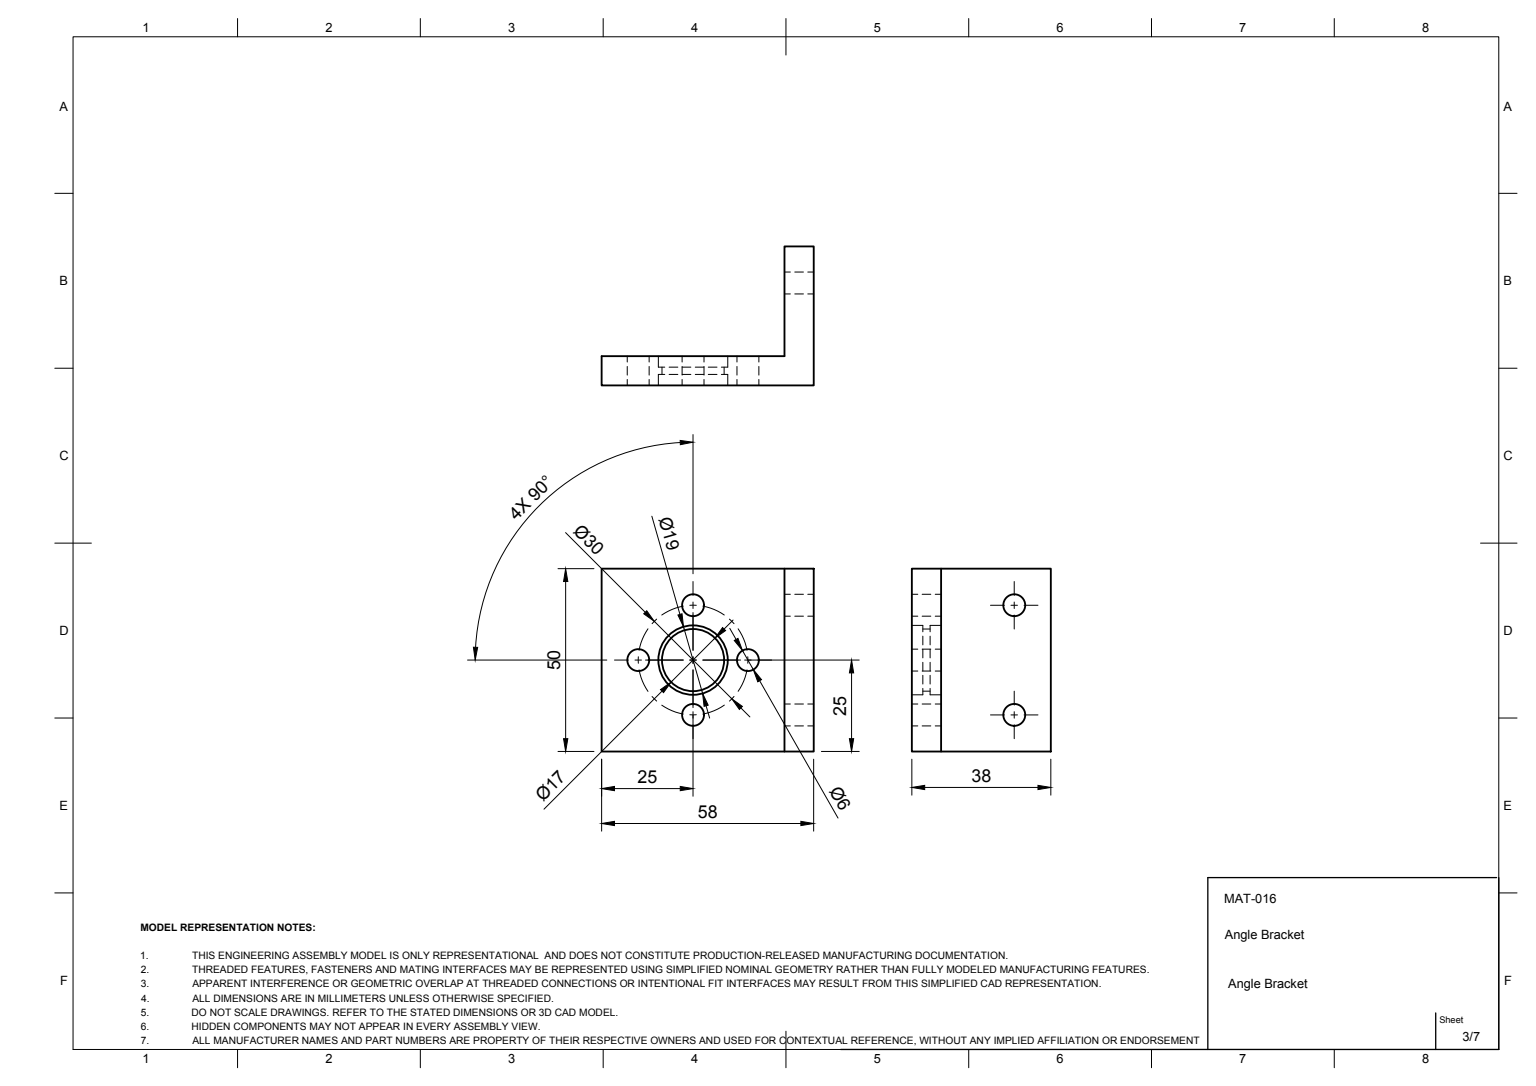
ISO-10303-21;
HEADER;
/* Generated by software containing ST-Developer
 * from STEP Tools, Inc. (www.steptools.com) 
 */

FILE_DESCRIPTION(
/* description */ ('STEP AP214'),
/* implementation_level */ '2;1');

FILE_NAME(
/* name */ 'Angle Bracket.step',
/* time_stamp */ '2026-11-14T06:10:26-08:00',
/* author */ (''),
/* organization */ (''),
/* preprocessor_version */ 'ST-DEVELOPER v20.2',
/* originating_system */ 'Autodesk Translation Framework v15.17.0.0',
/* authorisation */ '');

FILE_SCHEMA (('AUTOMOTIVE_DESIGN { 1 0 10303 214 3 1 1 }'));
ENDSEC;

DATA;
#10=MECHANICAL_DESIGN_GEOMETRIC_PRESENTATION_REPRESENTATION('',(#164),#10413);
#148=SHAPE_REPRESENTATION_RELATIONSHIP('SRR','None',#10453,#156);
#156=ADVANCED_BREP_SHAPE_REPRESENTATION('',(#172),#10405);
#164=STYLED_ITEM('',(#10502),#172);
#172=MANIFOLD_SOLID_BREP('Body1',#5299);
#180=FACE_BOUND('',#575,.T.);
#181=FACE_BOUND('',#576,.T.);
#182=FACE_BOUND('',#577,.T.);
#183=FACE_BOUND('',#578,.T.);
#184=FACE_BOUND('',#579,.T.);
#185=FACE_BOUND('',#581,.T.);
#186=FACE_BOUND('',#582,.T.);
#187=FACE_BOUND('',#583,.T.);
#188=FACE_BOUND('',#584,.T.);
#189=FACE_BOUND('',#585,.T.);
#190=FACE_BOUND('',#589,.T.);
#191=FACE_BOUND('',#591,.T.);
#192=FACE_BOUND('',#594,.T.);
#193=FACE_BOUND('',#595,.T.);
#194=FACE_BOUND('',#597,.T.);
#195=FACE_BOUND('',#598,.T.);
#219=PLANE('',#5425);
#220=PLANE('',#5426);
#221=PLANE('',#5427);
#222=PLANE('',#5428);
#223=PLANE('',#5429);
#224=PLANE('',#5430);
#225=PLANE('',#5431);
#226=PLANE('',#5432);
#227=PLANE('',#5433);
#228=PLANE('',#5434);
#275=FACE_OUTER_BOUND('',#565,.T.);
#276=FACE_OUTER_BOUND('',#566,.T.);
#277=FACE_OUTER_BOUND('',#567,.T.);
#278=FACE_OUTER_BOUND('',#568,.T.);
#279=FACE_OUTER_BOUND('',#569,.T.);
#280=FACE_OUTER_BOUND('',#570,.T.);
#281=FACE_OUTER_BOUND('',#571,.T.);
#282=FACE_OUTER_BOUND('',#572,.T.);
#283=FACE_OUTER_BOUND('',#573,.T.);
#284=FACE_OUTER_BOUND('',#574,.T.);
#285=FACE_OUTER_BOUND('',#580,.T.);
#286=FACE_OUTER_BOUND('',#586,.T.);
#287=FACE_OUTER_BOUND('',#587,.T.);
#288=FACE_OUTER_BOUND('',#588,.T.);
#289=FACE_OUTER_BOUND('',#590,.T.);
#290=FACE_OUTER_BOUND('',#592,.T.);
#291=FACE_OUTER_BOUND('',#593,.T.);
#292=FACE_OUTER_BOUND('',#596,.T.);
#293=FACE_OUTER_BOUND('',#599,.T.);
#565=EDGE_LOOP('',(#3222,#3223,#3224,#3225));
#566=EDGE_LOOP('',(#3226,#3227,#3228,#3229));
#567=EDGE_LOOP('',(#3230,#3231,#3232,#3233));
#568=EDGE_LOOP('',(#3234,#3235,#3236,#3237));
#569=EDGE_LOOP('',(#3238,#3239,#3240,#3241));
#570=EDGE_LOOP('',(#3242,#3243,#3244,#3245));
#571=EDGE_LOOP('',(#3246,#3247,#3248,#3249));
#572=EDGE_LOOP('',(#3250,#3251,#3252,#3253));
#573=EDGE_LOOP('',(#3254,#3255,#3256,#3257));
#574=EDGE_LOOP('',(#3258,#3259,#3260,#3261));
#575=EDGE_LOOP('',(#3262));
#576=EDGE_LOOP('',(#3263));
#577=EDGE_LOOP('',(#3264));
#578=EDGE_LOOP('',(#3265));
#579=EDGE_LOOP('',(#3266));
#580=EDGE_LOOP('',(#3267,#3268,#3269,#3270));
#581=EDGE_LOOP('',(#3271));
#582=EDGE_LOOP('',(#3272));
#583=EDGE_LOOP('',(#3273));
#584=EDGE_LOOP('',(#3274));
#585=EDGE_LOOP('',(#3275));
#586=EDGE_LOOP('',(#3276,#3277,#3278,#3279,#3280,#3281));
#587=EDGE_LOOP('',(#3282,#3283,#3284,#3285,#3286,#3287));
#588=EDGE_LOOP('',(#3288));
#589=EDGE_LOOP('',(#3289));
#590=EDGE_LOOP('',(#3290));
#591=EDGE_LOOP('',(#3291));
#592=EDGE_LOOP('',(#3292,#3293,#3294,#3295));
#593=EDGE_LOOP('',(#3296,#3297,#3298,#3299));
#594=EDGE_LOOP('',(#3300));
#595=EDGE_LOOP('',(#3301));
#596=EDGE_LOOP('',(#3302,#3303,#3304,#3305));
#597=EDGE_LOOP('',(#3306));
#598=EDGE_LOOP('',(#3307));
#599=EDGE_LOOP('',(#3308,#3309,#3310,#3311));
#894=LINE('',#7955,#1185);
#895=LINE('',#7961,#1186);
#896=LINE('',#7967,#1187);
#897=LINE('',#7973,#1188);
#898=LINE('',#7979,#1189);
#899=LINE('',#7985,#1190);
#900=LINE('',#7991,#1191);
#901=LINE('',#7997,#1192);
#902=LINE('',#8003,#1193);
#903=LINE('',#8008,#1194);
#904=LINE('',#8010,#1195);
#905=LINE('',#8012,#1196);
#906=LINE('',#8013,#1197);
#907=LINE('',#8017,#1198);
#908=LINE('',#8019,#1199);
#909=LINE('',#8021,#1200);
#910=LINE('',#8022,#1201);
#911=LINE('',#8024,#1202);
#912=LINE('',#8026,#1203);
#913=LINE('',#8028,#1204);
#914=LINE('',#8029,#1205);
#915=LINE('',#8031,#1206);
#916=LINE('',#8033,#1207);
#917=LINE('',#8035,#1208);
#918=LINE('',#8036,#1209);
#919=LINE('',#8041,#1210);
#920=LINE('',#8043,#1211);
#1185=VECTOR('',#6158,3.);
#1186=VECTOR('',#6165,3.);
#1187=VECTOR('',#6172,8.5);
#1188=VECTOR('',#6179,9.5);
#1189=VECTOR('',#6186,9.5);
#1190=VECTOR('',#6193,2.99999999999929);
#1191=VECTOR('',#6200,3.);
#1192=VECTOR('',#6207,2.99999999999976);
#1193=VECTOR('',#6214,3.);
#1194=VECTOR('',#6219,1000.);
#1195=VECTOR('',#6220,1000.);
#1196=VECTOR('',#6221,1000.);
#1197=VECTOR('',#6222,1000.);
#1198=VECTOR('',#6225,1000.);
#1199=VECTOR('',#6226,1000.);
#1200=VECTOR('',#6227,1000.);
#1201=VECTOR('',#6228,1000.);
#1202=VECTOR('',#6231,1000.);
#1203=VECTOR('',#6232,1000.);
#1204=VECTOR('',#6233,1000.);
#1205=VECTOR('',#6234,1000.);
#1206=VECTOR('',#6237,1000.);
#1207=VECTOR('',#6238,1000.);
#1208=VECTOR('',#6239,1000.);
#1209=VECTOR('',#6240,1000.);
#1210=VECTOR('',#6249,1000.);
#1211=VECTOR('',#6252,1000.);
#1476=CIRCLE('',#5399,3.);
#1477=CIRCLE('',#5400,3.);
#1478=CIRCLE('',#5402,3.);
#1479=CIRCLE('',#5403,3.);
#1480=CIRCLE('',#5405,8.5);
#1481=CIRCLE('',#5406,8.5);
#1482=CIRCLE('',#5408,9.5);
#1483=CIRCLE('',#5409,9.5);
#1484=CIRCLE('',#5411,9.5);
#1485=CIRCLE('',#5412,9.5);
#1486=CIRCLE('',#5414,2.99999999999929);
#1487=CIRCLE('',#5415,2.99999999999929);
#1488=CIRCLE('',#5417,3.);
#1489=CIRCLE('',#5418,3.);
#1490=CIRCLE('',#5420,2.99999999999976);
#1491=CIRCLE('',#5421,2.99999999999976);
#1492=CIRCLE('',#5423,3.);
#1493=CIRCLE('',#5424,3.);
#1917=VERTEX_POINT('',#7952);
#1918=VERTEX_POINT('',#7954);
#1919=VERTEX_POINT('',#7958);
#1920=VERTEX_POINT('',#7960);
#1921=VERTEX_POINT('',#7964);
#1922=VERTEX_POINT('',#7966);
#1923=VERTEX_POINT('',#7970);
#1924=VERTEX_POINT('',#7972);
#1925=VERTEX_POINT('',#7976);
#1926=VERTEX_POINT('',#7978);
#1927=VERTEX_POINT('',#7982);
#1928=VERTEX_POINT('',#7984);
#1929=VERTEX_POINT('',#7988);
#1930=VERTEX_POINT('',#7990);
#1931=VERTEX_POINT('',#7994);
#1932=VERTEX_POINT('',#7996);
#1933=VERTEX_POINT('',#8000);
#1934=VERTEX_POINT('',#8002);
#1935=VERTEX_POINT('',#8006);
#1936=VERTEX_POINT('',#8007);
#1937=VERTEX_POINT('',#8009);
#1938=VERTEX_POINT('',#8011);
#1939=VERTEX_POINT('',#8015);
#1940=VERTEX_POINT('',#8016);
#1941=VERTEX_POINT('',#8018);
#1942=VERTEX_POINT('',#8020);
#1943=VERTEX_POINT('',#8025);
#1944=VERTEX_POINT('',#8027);
#1945=VERTEX_POINT('',#8032);
#1946=VERTEX_POINT('',#8034);
#2436=EDGE_CURVE('',#1917,#1917,#1476,.T.);
#2437=EDGE_CURVE('',#1917,#1918,#894,.T.);
#2438=EDGE_CURVE('',#1918,#1918,#1477,.T.);
#2439=EDGE_CURVE('',#1919,#1919,#1478,.T.);
#2440=EDGE_CURVE('',#1919,#1920,#895,.T.);
#2441=EDGE_CURVE('',#1920,#1920,#1479,.T.);
#2442=EDGE_CURVE('',#1921,#1921,#1480,.T.);
#2443=EDGE_CURVE('',#1921,#1922,#896,.T.);
#2444=EDGE_CURVE('',#1922,#1922,#1481,.T.);
#2445=EDGE_CURVE('',#1923,#1923,#1482,.T.);
#2446=EDGE_CURVE('',#1923,#1924,#897,.T.);
#2447=EDGE_CURVE('',#1924,#1924,#1483,.T.);
#2448=EDGE_CURVE('',#1925,#1925,#1484,.T.);
#2449=EDGE_CURVE('',#1925,#1926,#898,.T.);
#2450=EDGE_CURVE('',#1926,#1926,#1485,.T.);
#2451=EDGE_CURVE('',#1927,#1927,#1486,.T.);
#2452=EDGE_CURVE('',#1927,#1928,#899,.T.);
#2453=EDGE_CURVE('',#1928,#1928,#1487,.T.);
#2454=EDGE_CURVE('',#1929,#1929,#1488,.T.);
#2455=EDGE_CURVE('',#1929,#1930,#900,.T.);
#2456=EDGE_CURVE('',#1930,#1930,#1489,.T.);
#2457=EDGE_CURVE('',#1931,#1931,#1490,.T.);
#2458=EDGE_CURVE('',#1931,#1932,#901,.T.);
#2459=EDGE_CURVE('',#1932,#1932,#1491,.T.);
#2460=EDGE_CURVE('',#1933,#1933,#1492,.T.);
#2461=EDGE_CURVE('',#1933,#1934,#902,.T.);
#2462=EDGE_CURVE('',#1934,#1934,#1493,.T.);
#2463=EDGE_CURVE('',#1935,#1936,#903,.T.);
#2464=EDGE_CURVE('',#1935,#1937,#904,.T.);
#2465=EDGE_CURVE('',#1938,#1937,#905,.T.);
#2466=EDGE_CURVE('',#1938,#1936,#906,.T.);
#2467=EDGE_CURVE('',#1939,#1940,#907,.T.);
#2468=EDGE_CURVE('',#1941,#1939,#908,.T.);
#2469=EDGE_CURVE('',#1942,#1941,#909,.T.);
#2470=EDGE_CURVE('',#1940,#1942,#910,.T.);
#2471=EDGE_CURVE('',#1940,#1938,#911,.T.);
#2472=EDGE_CURVE('',#1942,#1943,#912,.T.);
#2473=EDGE_CURVE('',#1944,#1943,#913,.T.);
#2474=EDGE_CURVE('',#1944,#1936,#914,.T.);
#2475=EDGE_CURVE('',#1939,#1937,#915,.T.);
#2476=EDGE_CURVE('',#1945,#1935,#916,.T.);
#2477=EDGE_CURVE('',#1946,#1945,#917,.T.);
#2478=EDGE_CURVE('',#1941,#1946,#918,.T.);
#2479=EDGE_CURVE('',#1943,#1946,#919,.T.);
#2480=EDGE_CURVE('',#1945,#1944,#920,.T.);
#3222=ORIENTED_EDGE('',*,*,#2436,.F.);
#3223=ORIENTED_EDGE('',*,*,#2437,.T.);
#3224=ORIENTED_EDGE('',*,*,#2438,.T.);
#3225=ORIENTED_EDGE('',*,*,#2437,.F.);
#3226=ORIENTED_EDGE('',*,*,#2439,.F.);
#3227=ORIENTED_EDGE('',*,*,#2440,.T.);
#3228=ORIENTED_EDGE('',*,*,#2441,.T.);
#3229=ORIENTED_EDGE('',*,*,#2440,.F.);
#3230=ORIENTED_EDGE('',*,*,#2442,.T.);
#3231=ORIENTED_EDGE('',*,*,#2443,.T.);
#3232=ORIENTED_EDGE('',*,*,#2444,.T.);
#3233=ORIENTED_EDGE('',*,*,#2443,.F.);
#3234=ORIENTED_EDGE('',*,*,#2445,.T.);
#3235=ORIENTED_EDGE('',*,*,#2446,.T.);
#3236=ORIENTED_EDGE('',*,*,#2447,.F.);
#3237=ORIENTED_EDGE('',*,*,#2446,.F.);
#3238=ORIENTED_EDGE('',*,*,#2448,.F.);
#3239=ORIENTED_EDGE('',*,*,#2449,.T.);
#3240=ORIENTED_EDGE('',*,*,#2450,.T.);
#3241=ORIENTED_EDGE('',*,*,#2449,.F.);
#3242=ORIENTED_EDGE('',*,*,#2451,.F.);
#3243=ORIENTED_EDGE('',*,*,#2452,.T.);
#3244=ORIENTED_EDGE('',*,*,#2453,.T.);
#3245=ORIENTED_EDGE('',*,*,#2452,.F.);
#3246=ORIENTED_EDGE('',*,*,#2454,.F.);
#3247=ORIENTED_EDGE('',*,*,#2455,.T.);
#3248=ORIENTED_EDGE('',*,*,#2456,.T.);
#3249=ORIENTED_EDGE('',*,*,#2455,.F.);
#3250=ORIENTED_EDGE('',*,*,#2457,.F.);
#3251=ORIENTED_EDGE('',*,*,#2458,.T.);
#3252=ORIENTED_EDGE('',*,*,#2459,.T.);
#3253=ORIENTED_EDGE('',*,*,#2458,.F.);
#3254=ORIENTED_EDGE('',*,*,#2460,.F.);
#3255=ORIENTED_EDGE('',*,*,#2461,.T.);
#3256=ORIENTED_EDGE('',*,*,#2462,.T.);
#3257=ORIENTED_EDGE('',*,*,#2461,.F.);
#3258=ORIENTED_EDGE('',*,*,#2463,.F.);
#3259=ORIENTED_EDGE('',*,*,#2464,.T.);
#3260=ORIENTED_EDGE('',*,*,#2465,.F.);
#3261=ORIENTED_EDGE('',*,*,#2466,.T.);
#3262=ORIENTED_EDGE('',*,*,#2462,.F.);
#3263=ORIENTED_EDGE('',*,*,#2459,.F.);
#3264=ORIENTED_EDGE('',*,*,#2456,.F.);
#3265=ORIENTED_EDGE('',*,*,#2453,.F.);
#3266=ORIENTED_EDGE('',*,*,#2450,.F.);
#3267=ORIENTED_EDGE('',*,*,#2467,.F.);
#3268=ORIENTED_EDGE('',*,*,#2468,.F.);
#3269=ORIENTED_EDGE('',*,*,#2469,.F.);
#3270=ORIENTED_EDGE('',*,*,#2470,.F.);
#3271=ORIENTED_EDGE('',*,*,#2460,.T.);
#3272=ORIENTED_EDGE('',*,*,#2457,.T.);
#3273=ORIENTED_EDGE('',*,*,#2454,.T.);
#3274=ORIENTED_EDGE('',*,*,#2451,.T.);
#3275=ORIENTED_EDGE('',*,*,#2447,.T.);
#3276=ORIENTED_EDGE('',*,*,#2466,.F.);
#3277=ORIENTED_EDGE('',*,*,#2471,.F.);
#3278=ORIENTED_EDGE('',*,*,#2470,.T.);
#3279=ORIENTED_EDGE('',*,*,#2472,.T.);
#3280=ORIENTED_EDGE('',*,*,#2473,.F.);
#3281=ORIENTED_EDGE('',*,*,#2474,.T.);
#3282=ORIENTED_EDGE('',*,*,#2468,.T.);
#3283=ORIENTED_EDGE('',*,*,#2475,.T.);
#3284=ORIENTED_EDGE('',*,*,#2464,.F.);
#3285=ORIENTED_EDGE('',*,*,#2476,.F.);
#3286=ORIENTED_EDGE('',*,*,#2477,.F.);
#3287=ORIENTED_EDGE('',*,*,#2478,.F.);
#3288=ORIENTED_EDGE('',*,*,#2448,.T.);
#3289=ORIENTED_EDGE('',*,*,#2444,.F.);
#3290=ORIENTED_EDGE('',*,*,#2445,.F.);
#3291=ORIENTED_EDGE('',*,*,#2442,.F.);
#3292=ORIENTED_EDGE('',*,*,#2467,.T.);
#3293=ORIENTED_EDGE('',*,*,#2471,.T.);
#3294=ORIENTED_EDGE('',*,*,#2465,.T.);
#3295=ORIENTED_EDGE('',*,*,#2475,.F.);
#3296=ORIENTED_EDGE('',*,*,#2478,.T.);
#3297=ORIENTED_EDGE('',*,*,#2479,.F.);
#3298=ORIENTED_EDGE('',*,*,#2472,.F.);
#3299=ORIENTED_EDGE('',*,*,#2469,.T.);
#3300=ORIENTED_EDGE('',*,*,#2436,.T.);
#3301=ORIENTED_EDGE('',*,*,#2439,.T.);
#3302=ORIENTED_EDGE('',*,*,#2463,.T.);
#3303=ORIENTED_EDGE('',*,*,#2474,.F.);
#3304=ORIENTED_EDGE('',*,*,#2480,.F.);
#3305=ORIENTED_EDGE('',*,*,#2476,.T.);
#3306=ORIENTED_EDGE('',*,*,#2438,.F.);
#3307=ORIENTED_EDGE('',*,*,#2441,.F.);
#3308=ORIENTED_EDGE('',*,*,#2479,.T.);
#3309=ORIENTED_EDGE('',*,*,#2477,.T.);
#3310=ORIENTED_EDGE('',*,*,#2480,.T.);
#3311=ORIENTED_EDGE('',*,*,#2473,.T.);
#4794=CYLINDRICAL_SURFACE('',#5398,3.);
#4795=CYLINDRICAL_SURFACE('',#5401,3.);
#4796=CYLINDRICAL_SURFACE('',#5404,8.5);
#4797=CYLINDRICAL_SURFACE('',#5407,9.5);
#4798=CYLINDRICAL_SURFACE('',#5410,9.5);
#4799=CYLINDRICAL_SURFACE('',#5413,2.99999999999929);
#4800=CYLINDRICAL_SURFACE('',#5416,3.);
#4801=CYLINDRICAL_SURFACE('',#5419,2.99999999999976);
#4802=CYLINDRICAL_SURFACE('',#5422,3.);
#5009=ADVANCED_FACE('',(#275),#4794,.F.);
#5010=ADVANCED_FACE('',(#276),#4795,.F.);
#5011=ADVANCED_FACE('',(#277),#4796,.F.);
#5012=ADVANCED_FACE('',(#278),#4797,.F.);
#5013=ADVANCED_FACE('',(#279),#4798,.F.);
#5014=ADVANCED_FACE('',(#280),#4799,.F.);
#5015=ADVANCED_FACE('',(#281),#4800,.F.);
#5016=ADVANCED_FACE('',(#282),#4801,.F.);
#5017=ADVANCED_FACE('',(#283),#4802,.F.);
#5018=ADVANCED_FACE('',(#284,#180,#181,#182,#183,#184),#219,.F.);
#5019=ADVANCED_FACE('',(#285,#185,#186,#187,#188,#189),#220,.T.);
#5020=ADVANCED_FACE('',(#286),#221,.F.);
#5021=ADVANCED_FACE('',(#287),#222,.F.);
#5022=ADVANCED_FACE('',(#288,#190),#223,.T.);
#5023=ADVANCED_FACE('',(#289,#191),#224,.T.);
#5024=ADVANCED_FACE('',(#290),#225,.F.);
#5025=ADVANCED_FACE('',(#291,#192,#193),#226,.T.);
#5026=ADVANCED_FACE('',(#292,#194,#195),#227,.F.);
#5027=ADVANCED_FACE('',(#293),#228,.F.);
#5299=CLOSED_SHELL('',(#5009,#5010,#5011,#5012,#5013,#5014,#5015,#5016,
#5017,#5018,#5019,#5020,#5021,#5022,#5023,#5024,#5025,#5026,#5027));
#5397=AXIS2_PLACEMENT_3D('',#7950,#6152,#6153);
#5398=AXIS2_PLACEMENT_3D('',#7951,#6154,#6155);
#5399=AXIS2_PLACEMENT_3D('',#7953,#6156,#6157);
#5400=AXIS2_PLACEMENT_3D('',#7956,#6159,#6160);
#5401=AXIS2_PLACEMENT_3D('',#7957,#6161,#6162);
#5402=AXIS2_PLACEMENT_3D('',#7959,#6163,#6164);
#5403=AXIS2_PLACEMENT_3D('',#7962,#6166,#6167);
#5404=AXIS2_PLACEMENT_3D('',#7963,#6168,#6169);
#5405=AXIS2_PLACEMENT_3D('',#7965,#6170,#6171);
#5406=AXIS2_PLACEMENT_3D('',#7968,#6173,#6174);
#5407=AXIS2_PLACEMENT_3D('',#7969,#6175,#6176);
#5408=AXIS2_PLACEMENT_3D('',#7971,#6177,#6178);
#5409=AXIS2_PLACEMENT_3D('',#7974,#6180,#6181);
#5410=AXIS2_PLACEMENT_3D('',#7975,#6182,#6183);
#5411=AXIS2_PLACEMENT_3D('',#7977,#6184,#6185);
#5412=AXIS2_PLACEMENT_3D('',#7980,#6187,#6188);
#5413=AXIS2_PLACEMENT_3D('',#7981,#6189,#6190);
#5414=AXIS2_PLACEMENT_3D('',#7983,#6191,#6192);
#5415=AXIS2_PLACEMENT_3D('',#7986,#6194,#6195);
#5416=AXIS2_PLACEMENT_3D('',#7987,#6196,#6197);
#5417=AXIS2_PLACEMENT_3D('',#7989,#6198,#6199);
#5418=AXIS2_PLACEMENT_3D('',#7992,#6201,#6202);
#5419=AXIS2_PLACEMENT_3D('',#7993,#6203,#6204);
#5420=AXIS2_PLACEMENT_3D('',#7995,#6205,#6206);
#5421=AXIS2_PLACEMENT_3D('',#7998,#6208,#6209);
#5422=AXIS2_PLACEMENT_3D('',#7999,#6210,#6211);
#5423=AXIS2_PLACEMENT_3D('',#8001,#6212,#6213);
#5424=AXIS2_PLACEMENT_3D('',#8004,#6215,#6216);
#5425=AXIS2_PLACEMENT_3D('',#8005,#6217,#6218);
#5426=AXIS2_PLACEMENT_3D('',#8014,#6223,#6224);
#5427=AXIS2_PLACEMENT_3D('',#8023,#6229,#6230);
#5428=AXIS2_PLACEMENT_3D('',#8030,#6235,#6236);
#5429=AXIS2_PLACEMENT_3D('',#8037,#6241,#6242);
#5430=AXIS2_PLACEMENT_3D('',#8038,#6243,#6244);
#5431=AXIS2_PLACEMENT_3D('',#8039,#6245,#6246);
#5432=AXIS2_PLACEMENT_3D('',#8040,#6247,#6248);
#5433=AXIS2_PLACEMENT_3D('',#8042,#6250,#6251);
#5434=AXIS2_PLACEMENT_3D('',#8044,#6253,#6254);
#6152=DIRECTION('axis',(0.,0.,1.));
#6153=DIRECTION('refdir',(1.,0.,0.));
#6154=DIRECTION('center_axis',(-1.,0.,0.));
#6155=DIRECTION('ref_axis',(0.,0.,1.));
#6156=DIRECTION('center_axis',(-1.,0.,0.));
#6157=DIRECTION('ref_axis',(0.,0.,1.));
#6158=DIRECTION('',(-1.,0.,0.));
#6159=DIRECTION('center_axis',(-1.,0.,0.));
#6160=DIRECTION('ref_axis',(0.,0.,1.));
#6161=DIRECTION('center_axis',(-1.,0.,0.));
#6162=DIRECTION('ref_axis',(0.,0.,1.));
#6163=DIRECTION('center_axis',(-1.,0.,0.));
#6164=DIRECTION('ref_axis',(0.,0.,1.));
#6165=DIRECTION('',(-1.,0.,0.));
#6166=DIRECTION('center_axis',(-1.,0.,0.));
#6167=DIRECTION('ref_axis',(0.,0.,1.));
#6168=DIRECTION('center_axis',(0.,0.,1.));
#6169=DIRECTION('ref_axis',(1.,0.,0.));
#6170=DIRECTION('center_axis',(0.,0.,-1.));
#6171=DIRECTION('ref_axis',(-1.,0.,0.));
#6172=DIRECTION('',(0.,0.,1.));
#6173=DIRECTION('center_axis',(0.,0.,1.));
#6174=DIRECTION('ref_axis',(1.,0.,0.));
#6175=DIRECTION('center_axis',(0.,0.,-1.));
#6176=DIRECTION('ref_axis',(-1.,0.,0.));
#6177=DIRECTION('center_axis',(0.,0.,1.));
#6178=DIRECTION('ref_axis',(1.,0.,0.));
#6179=DIRECTION('',(0.,0.,-1.));
#6180=DIRECTION('center_axis',(0.,0.,1.));
#6181=DIRECTION('ref_axis',(1.,0.,0.));
#6182=DIRECTION('center_axis',(0.,0.,1.));
#6183=DIRECTION('ref_axis',(1.,0.,0.));
#6184=DIRECTION('center_axis',(0.,0.,1.));
#6185=DIRECTION('ref_axis',(1.,0.,0.));
#6186=DIRECTION('',(0.,0.,1.));
#6187=DIRECTION('center_axis',(0.,0.,1.));
#6188=DIRECTION('ref_axis',(1.,0.,0.));
#6189=DIRECTION('center_axis',(0.,0.,1.));
#6190=DIRECTION('ref_axis',(1.,0.,0.));
#6191=DIRECTION('center_axis',(0.,0.,1.));
#6192=DIRECTION('ref_axis',(1.,0.,0.));
#6193=DIRECTION('',(0.,0.,1.));
#6194=DIRECTION('center_axis',(0.,0.,1.));
#6195=DIRECTION('ref_axis',(1.,0.,0.));
#6196=DIRECTION('center_axis',(0.,0.,1.));
#6197=DIRECTION('ref_axis',(1.,0.,0.));
#6198=DIRECTION('center_axis',(0.,0.,1.));
#6199=DIRECTION('ref_axis',(1.,0.,0.));
#6200=DIRECTION('',(0.,0.,1.));
#6201=DIRECTION('center_axis',(0.,0.,1.));
#6202=DIRECTION('ref_axis',(1.,0.,0.));
#6203=DIRECTION('center_axis',(0.,0.,1.));
#6204=DIRECTION('ref_axis',(1.,0.,0.));
#6205=DIRECTION('center_axis',(0.,0.,1.));
#6206=DIRECTION('ref_axis',(1.,0.,0.));
#6207=DIRECTION('',(0.,0.,1.));
#6208=DIRECTION('center_axis',(0.,0.,1.));
#6209=DIRECTION('ref_axis',(1.,0.,0.));
#6210=DIRECTION('center_axis',(0.,0.,1.));
#6211=DIRECTION('ref_axis',(1.,0.,0.));
#6212=DIRECTION('center_axis',(0.,0.,1.));
#6213=DIRECTION('ref_axis',(1.,0.,0.));
#6214=DIRECTION('',(0.,0.,1.));
#6215=DIRECTION('center_axis',(0.,0.,1.));
#6216=DIRECTION('ref_axis',(1.,0.,0.));
#6217=DIRECTION('center_axis',(0.,0.,-1.));
#6218=DIRECTION('ref_axis',(-1.,0.,0.));
#6219=DIRECTION('',(0.,-1.,0.));
#6220=DIRECTION('',(-1.,0.,0.));
#6221=DIRECTION('',(1.73472347597681E-17,1.,0.));
#6222=DIRECTION('',(1.,0.,0.));
#6223=DIRECTION('center_axis',(0.,0.,-1.));
#6224=DIRECTION('ref_axis',(-1.,0.,0.));
#6225=DIRECTION('',(-1.73472347597681E-17,-1.,0.));
#6226=DIRECTION('',(-1.,0.,0.));
#6227=DIRECTION('',(0.,1.,0.));
#6228=DIRECTION('',(1.,0.,0.));
#6229=DIRECTION('center_axis',(0.,1.,0.));
#6230=DIRECTION('ref_axis',(0.,0.,1.));
#6231=DIRECTION('',(0.,0.,1.));
#6232=DIRECTION('',(0.,0.,1.));
#6233=DIRECTION('',(1.,1.22464679914735E-16,0.));
#6234=DIRECTION('',(0.,0.,-1.));
#6235=DIRECTION('center_axis',(0.,-1.,0.));
#6236=DIRECTION('ref_axis',(0.,0.,-1.));
#6237=DIRECTION('',(0.,0.,1.));
#6238=DIRECTION('',(0.,0.,-1.));
#6239=DIRECTION('',(-1.,0.,0.));
#6240=DIRECTION('',(0.,0.,1.));
#6241=DIRECTION('center_axis',(0.,0.,1.));
#6242=DIRECTION('ref_axis',(1.,0.,0.));
#6243=DIRECTION('center_axis',(0.,0.,-1.));
#6244=DIRECTION('ref_axis',(1.,0.,0.));
#6245=DIRECTION('center_axis',(1.,-1.73472347597681E-17,0.));
#6246=DIRECTION('ref_axis',(1.73472347597681E-17,1.,0.));
#6247=DIRECTION('center_axis',(1.,0.,0.));
#6248=DIRECTION('ref_axis',(0.,0.,-1.));
#6249=DIRECTION('',(0.,1.,0.));
#6250=DIRECTION('center_axis',(1.,0.,0.));
#6251=DIRECTION('ref_axis',(0.,0.,-1.));
#6252=DIRECTION('',(0.,-1.,0.));
#6253=DIRECTION('center_axis',(0.,0.,-1.));
#6254=DIRECTION('ref_axis',(-1.,0.,0.));
#7950=CARTESIAN_POINT('',(0.,0.,0.));
#7951=CARTESIAN_POINT('Origin',(62.,10.,28.));
#7952=CARTESIAN_POINT('',(62.,10.,25.));
#7953=CARTESIAN_POINT('Origin',(62.,10.,28.));
#7954=CARTESIAN_POINT('',(54.,10.,25.));
#7955=CARTESIAN_POINT('',(62.,10.,25.));
#7956=CARTESIAN_POINT('Origin',(54.,10.,28.));
#7957=CARTESIAN_POINT('Origin',(62.,40.,28.));
#7958=CARTESIAN_POINT('',(62.,40.,25.));
#7959=CARTESIAN_POINT('Origin',(62.,40.,28.));
#7960=CARTESIAN_POINT('',(54.,40.,25.));
#7961=CARTESIAN_POINT('',(62.,40.,25.));
#7962=CARTESIAN_POINT('Origin',(54.,40.,28.));
#7963=CARTESIAN_POINT('Origin',(29.,24.9999999999997,2.));
#7964=CARTESIAN_POINT('',(20.5,24.9999999999997,3.));
#7965=CARTESIAN_POINT('Origin',(29.,24.9999999999997,3.));
#7966=CARTESIAN_POINT('',(20.5,24.9999999999997,5.));
#7967=CARTESIAN_POINT('',(20.5,24.9999999999997,2.));
#7968=CARTESIAN_POINT('Origin',(29.,24.9999999999997,5.));
#7969=CARTESIAN_POINT('Origin',(29.,24.9999999999997,3.));
#7970=CARTESIAN_POINT('',(38.5,24.9999999999997,3.));
#7971=CARTESIAN_POINT('Origin',(29.,24.9999999999997,3.));
#7972=CARTESIAN_POINT('',(38.5,24.9999999999997,0.));
#7973=CARTESIAN_POINT('',(38.5,24.9999999999997,3.));
#7974=CARTESIAN_POINT('Origin',(29.,24.9999999999997,0.));
#7975=CARTESIAN_POINT('Origin',(29.,24.9999999999997,5.));
#7976=CARTESIAN_POINT('',(19.5,24.9999999999997,5.));
#7977=CARTESIAN_POINT('Origin',(29.,24.9999999999997,5.));
#7978=CARTESIAN_POINT('',(19.5,24.9999999999997,8.));
#7979=CARTESIAN_POINT('',(19.5,24.9999999999997,5.));
#7980=CARTESIAN_POINT('Origin',(29.,24.9999999999997,8.));
#7981=CARTESIAN_POINT('Origin',(29.,10.,0.));
#7982=CARTESIAN_POINT('',(26.0000000000007,10.,0.));
#7983=CARTESIAN_POINT('Origin',(29.,10.,0.));
#7984=CARTESIAN_POINT('',(26.0000000000007,10.,8.));
#7985=CARTESIAN_POINT('',(26.0000000000007,10.,0.));
#7986=CARTESIAN_POINT('Origin',(29.,10.,8.));
#7987=CARTESIAN_POINT('Origin',(14.0000000000004,24.9999999999997,0.));
#7988=CARTESIAN_POINT('',(11.0000000000004,24.9999999999997,0.));
#7989=CARTESIAN_POINT('Origin',(14.0000000000004,24.9999999999997,0.));
#7990=CARTESIAN_POINT('',(11.0000000000004,24.9999999999997,8.));
#7991=CARTESIAN_POINT('',(11.0000000000004,24.9999999999997,0.));
#7992=CARTESIAN_POINT('Origin',(14.0000000000004,24.9999999999997,8.));
#7993=CARTESIAN_POINT('Origin',(44.,25.,0.));
#7994=CARTESIAN_POINT('',(41.0000000000002,25.,0.));
#7995=CARTESIAN_POINT('Origin',(44.,25.,0.));
#7996=CARTESIAN_POINT('',(41.0000000000002,25.,8.));
#7997=CARTESIAN_POINT('',(41.0000000000002,25.,0.));
#7998=CARTESIAN_POINT('Origin',(44.,25.,8.));
#7999=CARTESIAN_POINT('Origin',(29.,40.,0.));
#8000=CARTESIAN_POINT('',(26.,40.,0.));
#8001=CARTESIAN_POINT('Origin',(29.,40.,0.));
#8002=CARTESIAN_POINT('',(26.,40.,8.));
#8003=CARTESIAN_POINT('',(26.,40.,0.));
#8004=CARTESIAN_POINT('Origin',(29.,40.,8.));
#8005=CARTESIAN_POINT('Origin',(0.,0.,8.));
#8006=CARTESIAN_POINT('',(54.,50.,8.));
#8007=CARTESIAN_POINT('',(54.,-9.79717439317883E-16,8.));
#8008=CARTESIAN_POINT('',(54.,-9.79717439317883E-16,8.));
#8009=CARTESIAN_POINT('',(4.,50.,8.));
#8010=CARTESIAN_POINT('',(0.,50.,8.));
#8011=CARTESIAN_POINT('',(4.,0.,8.));
#8012=CARTESIAN_POINT('',(4.,50.,8.));
#8013=CARTESIAN_POINT('',(0.,0.,8.));
#8014=CARTESIAN_POINT('Origin',(0.,0.,0.));
#8015=CARTESIAN_POINT('',(4.,50.,0.));
#8016=CARTESIAN_POINT('',(4.,-6.93889390390723E-15,0.));
#8017=CARTESIAN_POINT('',(4.,-6.93889390390723E-17,0.));
#8018=CARTESIAN_POINT('',(62.,50.,0.));
#8019=CARTESIAN_POINT('',(0.,50.,0.));
#8020=CARTESIAN_POINT('',(62.,0.,0.));
#8021=CARTESIAN_POINT('',(62.,50.,0.));
#8022=CARTESIAN_POINT('',(0.,0.,0.));
#8023=CARTESIAN_POINT('Origin',(0.,0.,8.));
#8024=CARTESIAN_POINT('',(4.,-6.93889390390723E-15,-2.));
#8025=CARTESIAN_POINT('',(62.,0.,38.));
#8026=CARTESIAN_POINT('',(62.,0.,0.));
#8027=CARTESIAN_POINT('',(54.,-9.79717439317883E-16,38.));
#8028=CARTESIAN_POINT('',(62.,0.,38.));
#8029=CARTESIAN_POINT('',(54.,-9.79717439317883E-16,38.));
#8030=CARTESIAN_POINT('Origin',(0.,50.,8.));
#8031=CARTESIAN_POINT('',(4.,50.,-2.));
#8032=CARTESIAN_POINT('',(54.,50.,38.));
#8033=CARTESIAN_POINT('',(54.,50.,38.));
#8034=CARTESIAN_POINT('',(62.,50.,38.));
#8035=CARTESIAN_POINT('',(54.,50.,38.));
#8036=CARTESIAN_POINT('',(62.,50.,0.));
#8037=CARTESIAN_POINT('Origin',(29.,24.9999999999997,5.));
#8038=CARTESIAN_POINT('Origin',(29.,24.9999999999997,3.));
#8039=CARTESIAN_POINT('Origin',(4.,50.,-2.));
#8040=CARTESIAN_POINT('Origin',(62.,50.,0.));
#8041=CARTESIAN_POINT('',(62.,50.,38.));
#8042=CARTESIAN_POINT('Origin',(54.,-9.79717439317883E-16,38.));
#8043=CARTESIAN_POINT('',(54.,-9.79717439317883E-16,38.));
#8044=CARTESIAN_POINT('Origin',(0.,0.,38.));
#10395=UNCERTAINTY_MEASURE_WITH_UNIT(LENGTH_MEASURE(0.01),#10414,
'DISTANCE_ACCURACY_VALUE',
'Maximum model space distance between geometric entities at asserted c
onnectivities');
#10403=UNCERTAINTY_MEASURE_WITH_UNIT(LENGTH_MEASURE(0.01),#10414,
'DISTANCE_ACCURACY_VALUE',
'Maximum model space distance between geometric entities at asserted c
onnectivities');
#10405=(
GEOMETRIC_REPRESENTATION_CONTEXT(3)
GLOBAL_UNCERTAINTY_ASSIGNED_CONTEXT((#10395))
GLOBAL_UNIT_ASSIGNED_CONTEXT((#10414,#10416,#10417))
REPRESENTATION_CONTEXT('','3D')
);
#10413=(
GEOMETRIC_REPRESENTATION_CONTEXT(3)
GLOBAL_UNCERTAINTY_ASSIGNED_CONTEXT((#10403))
GLOBAL_UNIT_ASSIGNED_CONTEXT((#10414,#10416,#10417))
REPRESENTATION_CONTEXT('','3D')
);
#10414=(
LENGTH_UNIT()
NAMED_UNIT(*)
SI_UNIT(.MILLI.,.METRE.)
);
#10416=(
NAMED_UNIT(*)
PLANE_ANGLE_UNIT()
SI_UNIT($,.RADIAN.)
);
#10417=(
NAMED_UNIT(*)
SI_UNIT($,.STERADIAN.)
SOLID_ANGLE_UNIT()
);
#10419=SHAPE_DEFINITION_REPRESENTATION(#10428,#10453);
#10428=PRODUCT_DEFINITION_SHAPE('',$,#10463);
#10453=SHAPE_REPRESENTATION('',(#5397),#10405);
#10461=PRODUCT_DEFINITION_CONTEXT('part definition',#10490,'design');
#10463=PRODUCT_DEFINITION('Angle Bracket','Angle Bracket',#10472,#10461);
#10472=PRODUCT_DEFINITION_FORMATION('',$,#10493);
#10490=APPLICATION_CONTEXT(
'Core Data for Automotive Mechanical Design Process');
#10491=PRODUCT_CONTEXT('part definition',#10490,'mechanical');
#10493=PRODUCT('Angle Bracket','Angle Bracket',$,(#10491));
#10502=PRESENTATION_STYLE_ASSIGNMENT((#10506));
#10506=SURFACE_STYLE_USAGE(.BOTH.,#10510);
#10510=SURFACE_SIDE_STYLE('',(#10514));
#10514=SURFACE_STYLE_FILL_AREA(#10518);
#10518=FILL_AREA_STYLE('Opaque(61,176,222)',(#10522));
#10522=FILL_AREA_STYLE_COLOUR('Opaque(61,176,222)',#10526);
#10526=COLOUR_RGB('Opaque(61,176,222)',0.23921568627451,0.690196078431373,
0.870588235294118);
ENDSEC;
END-ISO-10303-21;
